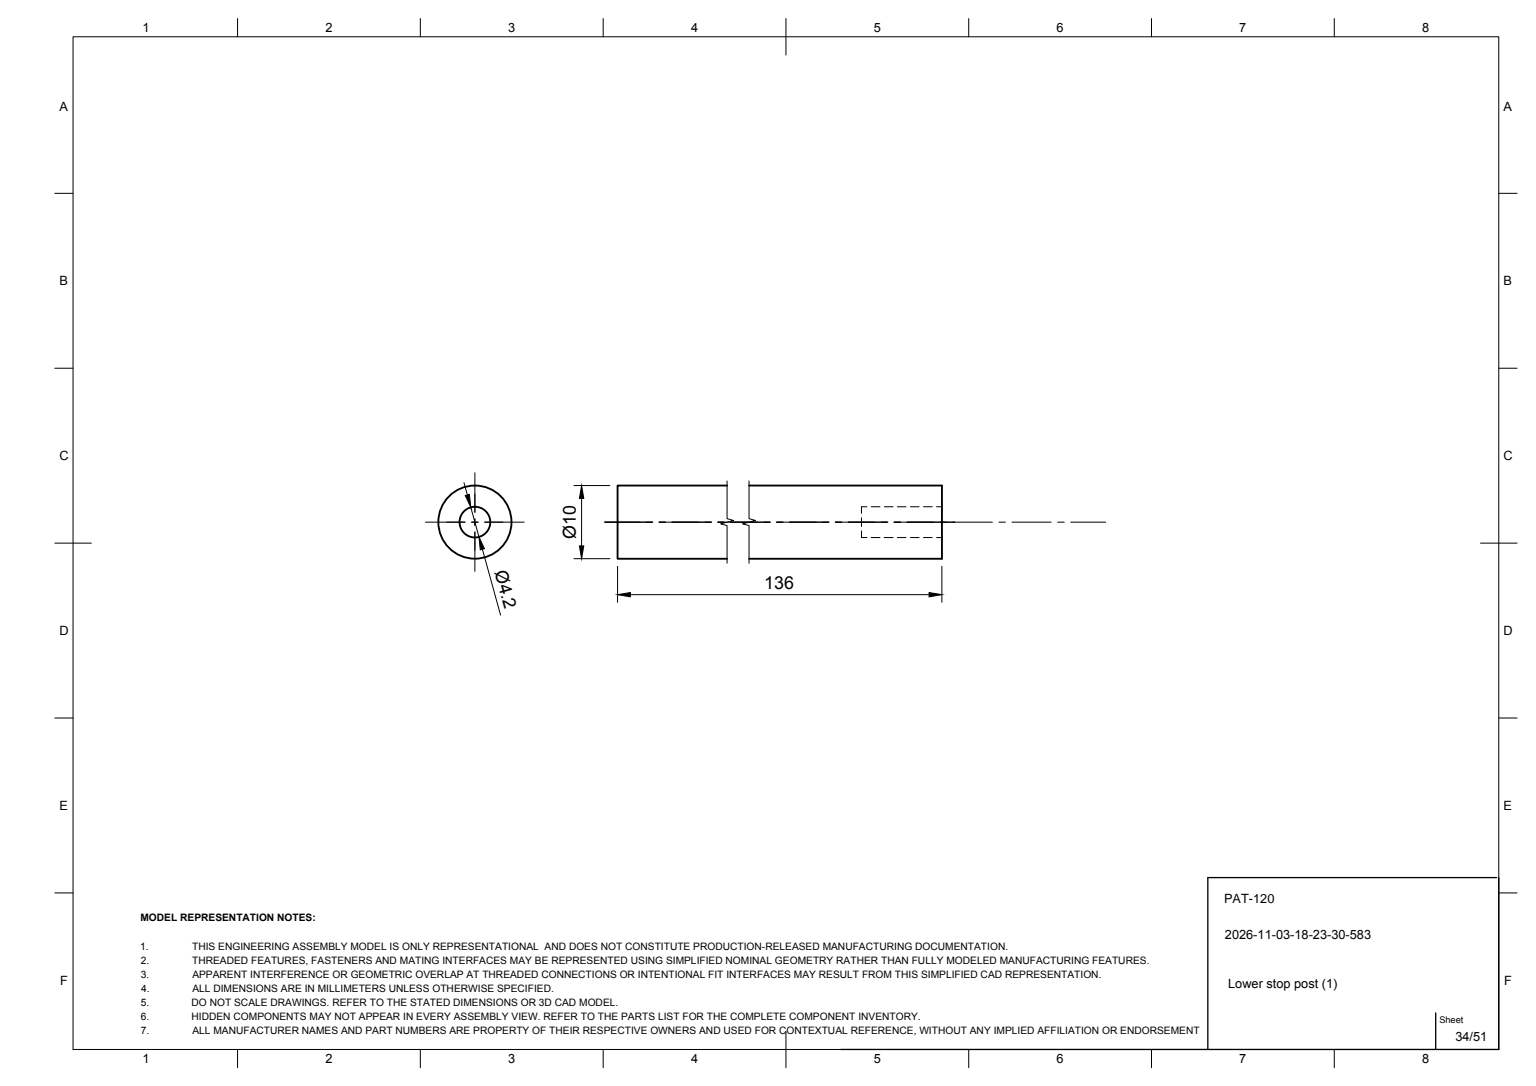
ISO-10303-21;
HEADER;
/* Generated by software containing ST-Developer
 * from STEP Tools, Inc. (www.steptools.com) 
 */

FILE_DESCRIPTION(
/* description */ ('Vibration shaker table dummy'),
/* implementation_level */ '2;1');

FILE_NAME(
/* name */ 'Lower stop post (1).step',
/* time_stamp */ '2026-10-27T10:55:14-07:00',
/* author */ (''),
/* organization */ (''),
/* preprocessor_version */ 'ST-DEVELOPER v20.2',
/* originating_system */ 'Autodesk Translation Framework v15.17.0.0',
/* authorisation */ '');

FILE_SCHEMA (('AUTOMOTIVE_DESIGN { 1 0 10303 214 3 1 1 }'));
ENDSEC;

DATA;
#10=MECHANICAL_DESIGN_GEOMETRIC_PRESENTATION_REPRESENTATION('',(#715),#22394);
#623=SHAPE_REPRESENTATION_RELATIONSHIP('SRR','None',#22669,#669);
#669=ADVANCED_BREP_SHAPE_REPRESENTATION('',(#761),#22375);
#715=STYLED_ITEM('',(#22947),#761);
#761=MANIFOLD_SOLID_BREP('Body1',#9233);
#945=FACE_BOUND('',#2290,.T.);
#1222=PLANE('',#10311);
#1223=PLANE('',#10315);
#1224=PLANE('',#10316);
#1617=FACE_OUTER_BOUND('',#2285,.T.);
#1618=FACE_OUTER_BOUND('',#2286,.T.);
#1619=FACE_OUTER_BOUND('',#2287,.T.);
#1620=FACE_OUTER_BOUND('',#2288,.T.);
#1621=FACE_OUTER_BOUND('',#2289,.T.);
#2285=EDGE_LOOP('',(#7458,#7459,#7460,#7461));
#2286=EDGE_LOOP('',(#7462));
#2287=EDGE_LOOP('',(#7463,#7464,#7465,#7466));
#2288=EDGE_LOOP('',(#7467));
#2289=EDGE_LOOP('',(#7468));
#2290=EDGE_LOOP('',(#7469));
#2980=LINE('',#21049,#3599);
#2981=LINE('',#21056,#3600);
#3599=VECTOR('',#12408,0.21);
#3600=VECTOR('',#12417,0.5);
#4104=CIRCLE('',#10309,0.21);
#4105=CIRCLE('',#10310,0.21);
#4106=CIRCLE('',#10313,0.5);
#4107=CIRCLE('',#10314,0.5);
#4771=VERTEX_POINT('',#21046);
#4772=VERTEX_POINT('',#21048);
#4773=VERTEX_POINT('',#21053);
#4774=VERTEX_POINT('',#21055);
#5722=EDGE_CURVE('',#4771,#4771,#4104,.T.);
#5723=EDGE_CURVE('',#4771,#4772,#2980,.T.);
#5724=EDGE_CURVE('',#4772,#4772,#4105,.T.);
#5725=EDGE_CURVE('',#4773,#4773,#4106,.T.);
#5726=EDGE_CURVE('',#4773,#4774,#2981,.T.);
#5727=EDGE_CURVE('',#4774,#4774,#4107,.T.);
#7458=ORIENTED_EDGE('',*,*,#5722,.F.);
#7459=ORIENTED_EDGE('',*,*,#5723,.T.);
#7460=ORIENTED_EDGE('',*,*,#5724,.T.);
#7461=ORIENTED_EDGE('',*,*,#5723,.F.);
#7462=ORIENTED_EDGE('',*,*,#5724,.F.);
#7463=ORIENTED_EDGE('',*,*,#5725,.F.);
#7464=ORIENTED_EDGE('',*,*,#5726,.T.);
#7465=ORIENTED_EDGE('',*,*,#5727,.T.);
#7466=ORIENTED_EDGE('',*,*,#5726,.F.);
#7467=ORIENTED_EDGE('',*,*,#5725,.T.);
#7468=ORIENTED_EDGE('',*,*,#5727,.F.);
#7469=ORIENTED_EDGE('',*,*,#5722,.T.);
#8616=CYLINDRICAL_SURFACE('',#10308,0.21);
#8617=CYLINDRICAL_SURFACE('',#10312,0.5);
#8982=ADVANCED_FACE('',(#1617),#8616,.F.);
#8983=ADVANCED_FACE('',(#1618),#1222,.F.);
#8984=ADVANCED_FACE('',(#1619),#8617,.T.);
#8985=ADVANCED_FACE('',(#1620),#1223,.T.);
#8986=ADVANCED_FACE('',(#1621,#945),#1224,.F.);
#9233=CLOSED_SHELL('',(#8982,#8983,#8984,#8985,#8986));
#10307=AXIS2_PLACEMENT_3D('',#21044,#12402,#12403);
#10308=AXIS2_PLACEMENT_3D('',#21045,#12404,#12405);
#10309=AXIS2_PLACEMENT_3D('',#21047,#12406,#12407);
#10310=AXIS2_PLACEMENT_3D('',#21050,#12409,#12410);
#10311=AXIS2_PLACEMENT_3D('',#21051,#12411,#12412);
#10312=AXIS2_PLACEMENT_3D('',#21052,#12413,#12414);
#10313=AXIS2_PLACEMENT_3D('',#21054,#12415,#12416);
#10314=AXIS2_PLACEMENT_3D('',#21057,#12418,#12419);
#10315=AXIS2_PLACEMENT_3D('',#21058,#12420,#12421);
#10316=AXIS2_PLACEMENT_3D('',#21059,#12422,#12423);
#12402=DIRECTION('axis',(0.,0.,1.));
#12403=DIRECTION('refdir',(1.,0.,0.));
#12404=DIRECTION('center_axis',(0.,0.,1.));
#12405=DIRECTION('ref_axis',(1.,0.,0.));
#12406=DIRECTION('center_axis',(0.,0.,1.));
#12407=DIRECTION('ref_axis',(1.,0.,0.));
#12408=DIRECTION('',(0.,0.,1.));
#12409=DIRECTION('center_axis',(0.,0.,1.));
#12410=DIRECTION('ref_axis',(1.,0.,0.));
#12411=DIRECTION('center_axis',(0.,0.,1.));
#12412=DIRECTION('ref_axis',(1.,0.,0.));
#12413=DIRECTION('center_axis',(0.,0.,1.));
#12414=DIRECTION('ref_axis',(1.,0.,0.));
#12415=DIRECTION('center_axis',(0.,0.,1.));
#12416=DIRECTION('ref_axis',(1.,0.,0.));
#12417=DIRECTION('',(0.,0.,-1.));
#12418=DIRECTION('center_axis',(0.,0.,1.));
#12419=DIRECTION('ref_axis',(1.,0.,0.));
#12420=DIRECTION('center_axis',(0.,0.,1.));
#12421=DIRECTION('ref_axis',(1.,0.,0.));
#12422=DIRECTION('center_axis',(0.,0.,1.));
#12423=DIRECTION('ref_axis',(1.,0.,0.));
#21044=CARTESIAN_POINT('',(0.,0.,0.));
#21045=CARTESIAN_POINT('Origin',(0.,6.,-0.1));
#21046=CARTESIAN_POINT('',(-0.21,6.,0.));
#21047=CARTESIAN_POINT('Origin',(0.,6.,0.));
#21048=CARTESIAN_POINT('',(-0.21,6.,1.1));
#21049=CARTESIAN_POINT('',(-0.21,6.,-0.1));
#21050=CARTESIAN_POINT('Origin',(0.,6.,1.1));
#21051=CARTESIAN_POINT('Origin',(0.,6.,1.1));
#21052=CARTESIAN_POINT('Origin',(0.,6.,0.));
#21053=CARTESIAN_POINT('',(-0.5,6.,13.6));
#21054=CARTESIAN_POINT('Origin',(0.,6.,13.6));
#21055=CARTESIAN_POINT('',(-0.5,6.,0.));
#21056=CARTESIAN_POINT('',(-0.5,6.,0.));
#21057=CARTESIAN_POINT('Origin',(0.,6.,0.));
#21058=CARTESIAN_POINT('Origin',(0.,6.,13.6));
#21059=CARTESIAN_POINT('Origin',(0.,6.,0.));
#22324=UNCERTAINTY_MEASURE_WITH_UNIT(LENGTH_MEASURE(0.001),#22395,
'DISTANCE_ACCURACY_VALUE',
'Maximum model space distance between geometric entities at asserted c
onnectivities');
#22343=UNCERTAINTY_MEASURE_WITH_UNIT(LENGTH_MEASURE(0.001),#22395,
'DISTANCE_ACCURACY_VALUE',
'Maximum model space distance between geometric entities at asserted c
onnectivities');
#22375=(
GEOMETRIC_REPRESENTATION_CONTEXT(3)
GLOBAL_UNCERTAINTY_ASSIGNED_CONTEXT((#22324))
GLOBAL_UNIT_ASSIGNED_CONTEXT((#22395,#22397,#22398))
REPRESENTATION_CONTEXT('','3D')
);
#22394=(
GEOMETRIC_REPRESENTATION_CONTEXT(3)
GLOBAL_UNCERTAINTY_ASSIGNED_CONTEXT((#22343))
GLOBAL_UNIT_ASSIGNED_CONTEXT((#22395,#22397,#22398))
REPRESENTATION_CONTEXT('','3D')
);
#22395=(
LENGTH_UNIT()
NAMED_UNIT(*)
SI_UNIT(.CENTI.,.METRE.)
);
#22397=(
NAMED_UNIT(*)
PLANE_ANGLE_UNIT()
SI_UNIT($,.RADIAN.)
);
#22398=(
NAMED_UNIT(*)
SI_UNIT($,.STERADIAN.)
SOLID_ANGLE_UNIT()
);
#22430=SHAPE_DEFINITION_REPRESENTATION(#22480,#22669);
#22480=PRODUCT_DEFINITION_SHAPE('',$,#22720);
#22669=SHAPE_REPRESENTATION('',(#10307),#22375);
#22688=PRODUCT_DEFINITION_CONTEXT('part definition',#22840,'design');
#22720=PRODUCT_DEFINITION('Lower stop post (1)','Lower stop post (1)',#22770,
#22688);
#22770=PRODUCT_DEFINITION_FORMATION('',$,#22873);
#22840=APPLICATION_CONTEXT(
'Core Data for Automotive Mechanical Design Process');
#22841=PRODUCT_CONTEXT('part definition',#22840,'mechanical');
#22873=PRODUCT('Lower stop post (1)','Lower stop post (1)',
'Lower stop post (1)',(#22841));
#22941=COLOUR_RGB('Light Blue',0.38,0.62,0.78);
#22942=FILL_AREA_STYLE_COLOUR('',#22941);
#22943=FILL_AREA_STYLE('',(#22942));
#22944=SURFACE_STYLE_FILL_AREA(#22943);
#22945=SURFACE_SIDE_STYLE('',(#22944));
#22946=SURFACE_STYLE_USAGE(.BOTH.,#22945);
#22947=PRESENTATION_STYLE_ASSIGNMENT((#22946));
ENDSEC;
END-ISO-10303-21;
